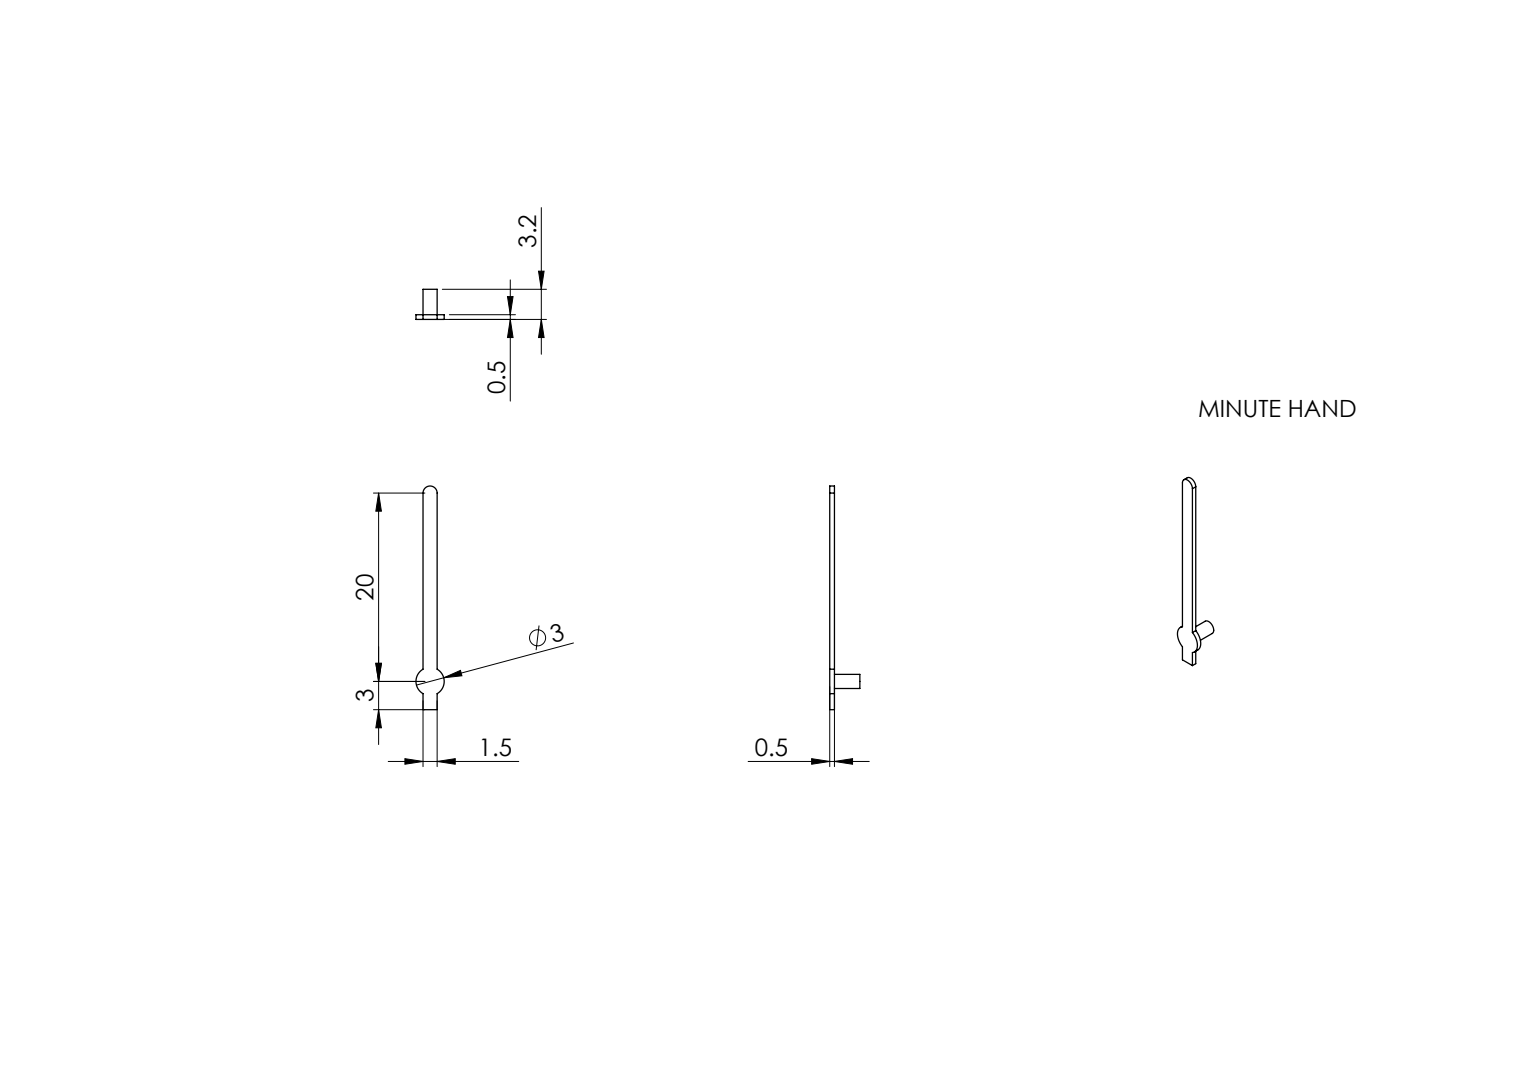
ISO-10303-21;
HEADER;
FILE_DESCRIPTION (('STEP AP214'),
    '1' );
FILE_NAME ('minute hand.step',
    '2026-10-26T11:20:31',
    ( '' ),
    ( '' ),
    'SwSTEP 2.0',
    'SolidWorks 2026',
    '' );
FILE_SCHEMA (( 'AUTOMOTIVE_DESIGN' ));
ENDSEC;

DATA;
#1=CARTESIAN_POINT ( 'NONE',  ( -0.7500000000000000000, 0.000000000000000000, 17.69999999999999929 ) ) ;
#7=ORIENTED_EDGE ( 'NONE', *, *, #1306, .T. ) ;
#18=DIRECTION ( 'NONE',  ( -0.000000000000000000, -0.000000000000000000, -1.000000000000000000 ) ) ;
#27=VERTEX_POINT ( 'NONE', #607 ) ;
#42=DIRECTION ( 'NONE',  ( 0.000000000000000000, 0.000000000000000000, 1.000000000000000000 ) ) ;
#70=ORIENTED_EDGE ( 'NONE', *, *, #687, .T. ) ;
#78=ORIENTED_EDGE ( 'NONE', *, *, #3001, .F. ) ;
#82=DIRECTION ( 'NONE',  ( 1.000000000000000000, 0.000000000000000000, 0.000000000000000000 ) ) ;
#87=LINE ( 'NONE', #2519, #444 ) ;
#97=CARTESIAN_POINT ( 'NONE',  ( 0.000000000000000000, 0.000000000000000000, 17.69999999999999929 ) ) ;
#113=ADVANCED_FACE ( 'NONE', ( #4266 ), #1343, .T. ) ;
#118=VECTOR ( 'NONE', #868, 1000.000000000000000 ) ;
#119=DIRECTION ( 'NONE',  ( 0.000000000000000000, 0.000000000000000000, 1.000000000000000000 ) ) ;
#140=DIRECTION ( 'NONE',  ( 0.000000000000000000, 0.000000000000000000, 1.000000000000000000 ) ) ;
#168=ORIENTED_EDGE ( 'NONE', *, *, #2422, .T. ) ;
#170=EDGE_LOOP ( 'NONE', ( #191, #1020, #400, #4142, #3752, #2488, #1167, #3281, #3139 ) ) ;
#183=DIRECTION ( 'NONE',  ( -1.000000000000000000, 0.000000000000000000, 0.000000000000000000 ) ) ;
#190=AXIS2_PLACEMENT_3D ( 'NONE', #1838, #4057, #3693 ) ;
#191=ORIENTED_EDGE ( 'NONE', *, *, #3421, .T. ) ;
#196=LINE ( 'NONE', #554, #4036 ) ;
#202=PLANE ( 'NONE',  #2959 ) ;
#256=FACE_OUTER_BOUND ( 'NONE', #2832, .T. ) ;
#258=ORIENTED_EDGE ( 'NONE', *, *, #4554, .T. ) ;
#260=AXIS2_PLACEMENT_3D ( 'NONE', #4512, #2060, #1677 ) ;
#292=CARTESIAN_POINT ( 'NONE',  ( -0.7500000000000001110, 20.00000000000000000, 18.19999999999999929 ) ) ;
#313=DIRECTION ( 'NONE',  ( 1.000000000000000000, 0.000000000000000000, 0.000000000000000000 ) ) ;
#316=DIRECTION ( 'NONE',  ( 0.000000000000000000, 0.000000000000000000, -1.000000000000000000 ) ) ;
#370=FACE_OUTER_BOUND ( 'NONE', #716, .T. ) ;
#386=ADVANCED_FACE ( 'NONE', ( #370 ), #2455, .F. ) ;
#396=DIRECTION ( 'NONE',  ( 1.000000000000000000, 0.000000000000000000, -0.000000000000000000 ) ) ;
#399=ORIENTED_EDGE ( 'NONE', *, *, #2054, .T. ) ;
#400=ORIENTED_EDGE ( 'NONE', *, *, #1846, .F. ) ;
#402=CARTESIAN_POINT ( 'NONE',  ( 0.7500000000000000000, -2.999999999999999556, 17.69999999999999929 ) ) ;
#416=FACE_OUTER_BOUND ( 'NONE', #1243, .T. ) ;
#419=CARTESIAN_POINT ( 'NONE',  ( 0.7500000000000001110, 1.299038105676658450, 17.69999999999999929 ) ) ;
#435=DIRECTION ( 'NONE',  ( -1.000000000000000000, 0.000000000000000000, -0.000000000000000000 ) ) ;
#443=ORIENTED_EDGE ( 'NONE', *, *, #2740, .F. ) ;
#444=VECTOR ( 'NONE', #4378, 1000.000000000000000 ) ;
#449=ORIENTED_EDGE ( 'NONE', *, *, #3217, .T. ) ;
#453=UNCERTAINTY_MEASURE_WITH_UNIT (LENGTH_MEASURE( 1.000000000000000082E-05 ), #1801, 'distance_accuracy_value', 'NONE');
#477=VERTEX_POINT ( 'NONE', #2505 ) ;
#478=ORIENTED_EDGE ( 'NONE', *, *, #3950, .F. ) ;
#482=LINE ( 'NONE', #3407, #3156 ) ;
#510=CARTESIAN_POINT ( 'NONE',  ( 0.7500000000000001110, 20.00000000000000000, 17.69999999999999929 ) ) ;
#511=LINE ( 'NONE', #1671, #1812 ) ;
#512=CARTESIAN_POINT ( 'NONE',  ( 0.000000000000000000, 20.00000000000000000, 17.69999999999999929 ) ) ;
#516=EDGE_CURVE ( 'NONE', #1550, #1737, #1460, .T. ) ;
#521=CARTESIAN_POINT ( 'NONE',  ( 0.7500000000000000000, -2.999999999999999556, 17.69999999999999929 ) ) ;
#524=ORIENTED_EDGE ( 'NONE', *, *, #4465, .F. ) ;
#541=CARTESIAN_POINT ( 'NONE',  ( 0.000000000000000000, 0.000000000000000000, 18.19999999999999929 ) ) ;
#544=DIRECTION ( 'NONE',  ( 0.000000000000000000, 0.000000000000000000, 1.000000000000000000 ) ) ;
#554=CARTESIAN_POINT ( 'NONE',  ( -0.7500000000000001110, 1.299038105676658450, 17.69999999999999929 ) ) ;
#556=ORIENTED_EDGE ( 'NONE', *, *, #1846, .T. ) ;
#562=ADVANCED_FACE ( 'NONE', ( #416 ), #2265, .T. ) ;
#566=AXIS2_PLACEMENT_3D ( 'NONE', #1204, #140, #4135 ) ;
#570=ORIENTED_EDGE ( 'NONE', *, *, #2926, .T. ) ;
#607=CARTESIAN_POINT ( 'NONE',  ( 0.7500000000000000000, -1.299038105676658450, 18.19999999999999929 ) ) ;
#635=CIRCLE ( 'NONE', #3283, 1.500000000000000222 ) ;
#658=VECTOR ( 'NONE', #781, 1000.000000000000000 ) ;
#677=CIRCLE ( 'NONE', #3941, 1.500000000000000222 ) ;
#678=DIRECTION ( 'NONE',  ( 0.000000000000000000, 0.000000000000000000, 1.000000000000000000 ) ) ;
#687=EDGE_CURVE ( 'NONE', #1161, #2307, #2576, .T. ) ;
#699=DIRECTION ( 'NONE',  ( 0.000000000000000000, 0.000000000000000000, 1.000000000000000000 ) ) ;
#714=DIRECTION ( 'NONE',  ( 0.000000000000000000, 0.000000000000000000, 1.000000000000000000 ) ) ;
#715=VERTEX_POINT ( 'NONE', #3488 ) ;
#716=EDGE_LOOP ( 'NONE', ( #908, #4000 ) ) ;
#720=ORIENTED_EDGE ( 'NONE', *, *, #4282, .F. ) ;
#723=DIRECTION ( 'NONE',  ( 0.000000000000000000, 0.000000000000000000, 1.000000000000000000 ) ) ;
#753=SHAPE_DEFINITION_REPRESENTATION ( #1564, #773 ) ;
#755=DIRECTION ( 'NONE',  ( -1.000000000000000000, 0.000000000000000000, 0.000000000000000000 ) ) ;
#756=CARTESIAN_POINT ( 'NONE',  ( 0.7500000000000001110, 9.184850993605150903E-17, 15.00000000000000178 ) ) ;
#765=VERTEX_POINT ( 'NONE', #1699 ) ;
#773=SHAPE_REPRESENTATION ( 'minute hand', ( #2928 ), #3769 ) ;
#774=FACE_OUTER_BOUND ( 'NONE', #4403, .T. ) ;
#781=DIRECTION ( 'NONE',  ( 0.000000000000000000, 0.000000000000000000, 1.000000000000000000 ) ) ;
#788=VERTEX_POINT ( 'NONE', #975 ) ;
#805=PLANE ( 'NONE',  #1597 ) ;
#809=CARTESIAN_POINT ( 'NONE',  ( -0.7500000000000001110, 20.00000000000000000, 17.69999999999999929 ) ) ;
#820=ADVANCED_FACE ( 'NONE', ( #2331 ), #3803, .T. ) ;
#837=UNCERTAINTY_MEASURE_WITH_UNIT (LENGTH_MEASURE( 1.000000000000000082E-05 ), #4288, 'distance_accuracy_value', 'NONE');
#848=AXIS2_PLACEMENT_3D ( 'NONE', #3084, #1630, #544 ) ;
#868=DIRECTION ( 'NONE',  ( -0.000000000000000000, -0.000000000000000000, -1.000000000000000000 ) ) ;
#908=ORIENTED_EDGE ( 'NONE', *, *, #3418, .F. ) ;
#911=DIRECTION ( 'NONE',  ( -0.000000000000000000, -0.000000000000000000, -1.000000000000000000 ) ) ;
#933=ORIENTED_EDGE ( 'NONE', *, *, #4502, .F. ) ;
#951=PLANE ( 'NONE',  #848 ) ;
#975=CARTESIAN_POINT ( 'NONE',  ( -0.7500000000000000000, -1.299038105676658450, 18.19999999999999929 ) ) ;
#990=DIRECTION ( 'NONE',  ( -0.000000000000000000, -1.000000000000000000, 0.000000000000000000 ) ) ;
#1000=ORIENTED_EDGE ( 'NONE', *, *, #3421, .F. ) ;
#1006=CIRCLE ( 'NONE', #3202, 1.500000000000000222 ) ;
#1018=LINE ( 'NONE', #3627, #2450 ) ;
#1020=ORIENTED_EDGE ( 'NONE', *, *, #3950, .T. ) ;
#1023=DIRECTION ( 'NONE',  ( -1.000000000000000000, 0.000000000000000000, 0.000000000000000000 ) ) ;
#1059=ADVANCED_FACE ( 'NONE', ( #2531 ), #3958, .T. ) ;
#1071=ORIENTED_EDGE ( 'NONE', *, *, #2422, .F. ) ;
#1096=CIRCLE ( 'NONE', #3147, 0.7500000000000001110 ) ;
#1126=CARTESIAN_POINT ( 'NONE',  ( 0.7500000000000001110, 1.299038105676658450, 17.69999999999999929 ) ) ;
#1161=VERTEX_POINT ( 'NONE', #809 ) ;
#1167=ORIENTED_EDGE ( 'NONE', *, *, #2110, .T. ) ;
#1203=ADVANCED_BREP_SHAPE_REPRESENTATION ( '', ( #1412, #2928 ), #3769 ) ;
#1204=CARTESIAN_POINT ( 'NONE',  ( 0.000000000000000000, 0.000000000000000000, 17.69999999999999929 ) ) ;
#1207=ORIENTED_EDGE ( 'NONE', *, *, #687, .F. ) ;
#1225=FACE_OUTER_BOUND ( 'NONE', #1963, .T. ) ;
#1226=CARTESIAN_POINT ( 'NONE',  ( 0.7500000000000001110, 9.184850993605150903E-17, 17.69999999999999929 ) ) ;
#1243=EDGE_LOOP ( 'NONE', ( #4067, #570, #933, #1367 ) ) ;
#1261=AXIS2_PLACEMENT_3D ( 'NONE', #2615, #3685, #2908 ) ;
#1270=VERTEX_POINT ( 'NONE', #4177 ) ;
#1273=VECTOR ( 'NONE', #3225, 1000.000000000000000 ) ;
#1278=DIRECTION ( 'NONE',  ( -0.000000000000000000, -1.000000000000000000, -0.000000000000000000 ) ) ;
#1295=LINE ( 'NONE', #3165, #2483 ) ;
#1299=EDGE_LOOP ( 'NONE', ( #1806, #4350, #399, #3813 ) ) ;
#1306=EDGE_CURVE ( 'NONE', #715, #1870, #196, .T. ) ;
#1320=SURFACE_STYLE_USAGE ( .BOTH. , #3761 ) ;
#1323=DIRECTION ( 'NONE',  ( 0.000000000000000000, 0.000000000000000000, 1.000000000000000000 ) ) ;
#1326=LINE ( 'NONE', #2372, #1627 ) ;
#1342=VECTOR ( 'NONE', #3381, 1000.000000000000000 ) ;
#1343=PLANE ( 'NONE',  #4188 ) ;
#1358=ORIENTED_EDGE ( 'NONE', *, *, #4137, .F. ) ;
#1367=ORIENTED_EDGE ( 'NONE', *, *, #4282, .T. ) ;
#1369=DIRECTION ( 'NONE',  ( -0.000000000000000000, -1.000000000000000000, 0.000000000000000000 ) ) ;
#1372=LINE ( 'NONE', #3247, #2978 ) ;
#1412=MANIFOLD_SOLID_BREP ( 'Extrude-Thin1', #2143 ) ;
#1445=( NAMED_UNIT ( * ) PLANE_ANGLE_UNIT ( ) SI_UNIT ( $, .RADIAN. ) );
#1460=LINE ( 'NONE', #1, #1273 ) ;
#1508=ORIENTED_EDGE ( 'NONE', *, *, #3086, .T. ) ;
#1526=ADVANCED_FACE ( 'NONE', ( #4069, #1823 ), #805, .F. ) ;
#1541=EDGE_LOOP ( 'NONE', ( #3473, #2533, #2637, #3666 ) ) ;
#1544=ORIENTED_EDGE ( 'NONE', *, *, #2306, .T. ) ;
#1550=VERTEX_POINT ( 'NONE', #1847 ) ;
#1560=VERTEX_POINT ( 'NONE', #419 ) ;
#1564=PRODUCT_DEFINITION_SHAPE ( 'NONE', 'NONE',  #3507 ) ;
#1570=ORIENTED_EDGE ( 'NONE', *, *, #516, .T. ) ;
#1590=ORIENTED_EDGE ( 'NONE', *, *, #2926, .F. ) ;
#1597=AXIS2_PLACEMENT_3D ( 'NONE', #97, #119, #396 ) ;
#1606=VECTOR ( 'NONE', #2974, 1000.000000000000000 ) ;
#1627=VECTOR ( 'NONE', #1278, 1000.000000000000000 ) ;
#1630=DIRECTION ( 'NONE',  ( 0.000000000000000000, 1.000000000000000000, -0.000000000000000000 ) ) ;
#1631=DIRECTION ( 'NONE',  ( 0.000000000000000000, 0.000000000000000000, 1.000000000000000000 ) ) ;
#1638=CARTESIAN_POINT ( 'NONE',  ( -0.7500000000000001110, 0.000000000000000000, 18.19999999999999929 ) ) ;
#1648=DIRECTION ( 'NONE',  ( 0.000000000000000000, 0.000000000000000000, 1.000000000000000000 ) ) ;
#1665=LINE ( 'NONE', #2004, #1342 ) ;
#1669=CARTESIAN_POINT ( 'NONE',  ( 0.000000000000000000, 0.000000000000000000, 17.69999999999999929 ) ) ;
#1670=ADVANCED_FACE ( 'NONE', ( #4567 ), #951, .F. ) ;
#1671=CARTESIAN_POINT ( 'NONE',  ( -0.7500000000000000000, -2.999999999999999556, 17.69999999999999929 ) ) ;
#1677=DIRECTION ( 'NONE',  ( -0.000000000000000000, 0.000000000000000000, 1.000000000000000000 ) ) ;
#1680=CYLINDRICAL_SURFACE ( 'NONE', #3112, 1.500000000000000222 ) ;
#1697=CARTESIAN_POINT ( 'NONE',  ( 0.7500000000000001110, 0.000000000000000000, 17.69999999999999929 ) ) ;
#1699=CARTESIAN_POINT ( 'NONE',  ( 0.7500000000000001110, 1.299038105676658450, 18.19999999999999929 ) ) ;
#1705=DIRECTION ( 'NONE',  ( 0.000000000000000000, 0.000000000000000000, 1.000000000000000000 ) ) ;
#1712=DIRECTION ( 'NONE',  ( 0.000000000000000000, 0.000000000000000000, 1.000000000000000000 ) ) ;
#1737=VERTEX_POINT ( 'NONE', #3177 ) ;
#1738=DIRECTION ( 'NONE',  ( 1.000000000000000000, 0.000000000000000000, -0.000000000000000000 ) ) ;
#1739=CARTESIAN_POINT ( 'NONE',  ( 0.000000000000000000, 0.000000000000000000, 17.69999999999999929 ) ) ;
#1753=DIRECTION ( 'NONE',  ( 1.000000000000000000, 0.000000000000000000, -0.000000000000000000 ) ) ;
#1767=CIRCLE ( 'NONE', #3822, 0.7500000000000001110 ) ;
#1768=EDGE_CURVE ( 'NONE', #4595, #1560, #1006, .T. ) ;
#1780=CARTESIAN_POINT ( 'NONE',  ( 0.000000000000000000, 0.000000000000000000, 0.000000000000000000 ) ) ;
#1786=CARTESIAN_POINT ( 'NONE',  ( 0.7500000000000000000, 0.000000000000000000, 18.19999999999999929 ) ) ;
#1801=( LENGTH_UNIT ( ) NAMED_UNIT ( * ) SI_UNIT ( .MILLI., .METRE. ) );
#1806=ORIENTED_EDGE ( 'NONE', *, *, #1935, .F. ) ;
#1812=VECTOR ( 'NONE', #2741, 1000.000000000000000 ) ;
#1820=EDGE_LOOP ( 'NONE', ( #556, #2302, #1358, #168 ) ) ;
#1822=ORIENTED_EDGE ( 'NONE', *, *, #4059, .F. ) ;
#1823=FACE_BOUND ( 'NONE', #4209, .T. ) ;
#1838=CARTESIAN_POINT ( 'NONE',  ( 0.000000000000000000, 0.000000000000000000, 18.19999999999999929 ) ) ;
#1846=EDGE_CURVE ( 'NONE', #3324, #477, #1372, .T. ) ;
#1847=CARTESIAN_POINT ( 'NONE',  ( -0.7500000000000000000, -1.299038105676658450, 17.69999999999999929 ) ) ;
#1870=VERTEX_POINT ( 'NONE', #4038 ) ;
#1886=DIRECTION ( 'NONE',  ( -0.000000000000000000, 0.000000000000000000, 1.000000000000000000 ) ) ;
#1918=VECTOR ( 'NONE', #3458, 1000.000000000000000 ) ;
#1934=ORIENTED_EDGE ( 'NONE', *, *, #2690, .F. ) ;
#1935=EDGE_CURVE ( 'NONE', #1560, #765, #2953, .T. ) ;
#1962=DIRECTION ( 'NONE',  ( -0.000000000000000000, -0.000000000000000000, -1.000000000000000000 ) ) ;
#1963=EDGE_LOOP ( 'NONE', ( #3306, #1934, #1207, #4237 ) ) ;
#1984=LINE ( 'NONE', #2006, #1918 ) ;
#1990=DIRECTION ( 'NONE',  ( -0.000000000000000000, -0.000000000000000000, -1.000000000000000000 ) ) ;
#2001=CARTESIAN_POINT ( 'NONE',  ( 0.000000000000000000, 0.000000000000000000, 18.19999999999999929 ) ) ;
#2004=CARTESIAN_POINT ( 'NONE',  ( 0.7500000000000001110, 0.000000000000000000, 17.69999999999999929 ) ) ;
#2006=CARTESIAN_POINT ( 'NONE',  ( 0.7500000000000001110, 0.000000000000000000, 18.19999999999999929 ) ) ;
#2008=CARTESIAN_POINT ( 'NONE',  ( -0.7500000000000001110, 0.000000000000000000, 15.00000000000000178 ) ) ;
#2033=PRODUCT_DEFINITION_FORMATION_WITH_SPECIFIED_SOURCE ( 'ANY', '', #2787, .NOT_KNOWN. ) ;
#2048=DIRECTION ( 'NONE',  ( -0.000000000000000000, -0.000000000000000000, -1.000000000000000000 ) ) ;
#2054=EDGE_CURVE ( 'NONE', #2878, #1270, #2643, .T. ) ;
#2060=DIRECTION ( 'NONE',  ( -1.000000000000000000, 0.000000000000000000, -0.000000000000000000 ) ) ;
#2069=CYLINDRICAL_SURFACE ( 'NONE', #4016, 0.7500000000000001110 ) ;
#2071=( NAMED_UNIT ( * ) PLANE_ANGLE_UNIT ( ) SI_UNIT ( $, .RADIAN. ) );
#2079=LINE ( 'NONE', #2401, #3946 ) ;
#2080=CARTESIAN_POINT ( 'NONE',  ( -0.7500000000000000000, 0.000000000000000000, 18.19999999999999929 ) ) ;
#2110=EDGE_CURVE ( 'NONE', #765, #1270, #1984, .T. ) ;
#2123=CIRCLE ( 'NONE', #4319, 0.7500000000000001110 ) ;
#2138=DIRECTION ( 'NONE',  ( 1.000000000000000000, 0.000000000000000000, 0.000000000000000000 ) ) ;
#2143=CLOSED_SHELL ( 'NONE', ( #820, #562, #3805, #2749, #113, #386, #1526, #3104, #1059, #2895, #3414, #2984, #3887, #1670 ) ) ;
#2145=LINE ( 'NONE', #402, #3166 ) ;
#2153=CARTESIAN_POINT ( 'NONE',  ( 0.000000000000000000, 20.00000000000000000, 18.19999999999999929 ) ) ;
#2214=EDGE_CURVE ( 'NONE', #4100, #4120, #1767, .T. ) ;
#2231=CARTESIAN_POINT ( 'NONE',  ( 0.000000000000000000, 0.000000000000000000, 18.19999999999999929 ) ) ;
#2234=CIRCLE ( 'NONE', #2848, 1.500000000000000222 ) ;
#2253=ORIENTED_EDGE ( 'NONE', *, *, #2054, .F. ) ;
#2261=CARTESIAN_POINT ( 'NONE',  ( 0.7500000000000000000, -2.999999999999999556, 17.69999999999999929 ) ) ;
#2262=AXIS2_PLACEMENT_3D ( 'NONE', #1697, #3573, #316 ) ;
#2265=CYLINDRICAL_SURFACE ( 'NONE', #2857, 1.500000000000000222 ) ;
#2302=ORIENTED_EDGE ( 'NONE', *, *, #3086, .F. ) ;
#2306=EDGE_CURVE ( 'NONE', #1870, #1550, #2981, .T. ) ;
#2307=VERTEX_POINT ( 'NONE', #292 ) ;
#2316=EDGE_LOOP ( 'NONE', ( #2732, #3638, #3020, #4066, #3679, #2871, #3812, #3526, #2804 ) ) ;
#2323=DIRECTION ( 'NONE',  ( 0.000000000000000000, 0.000000000000000000, 1.000000000000000000 ) ) ;
#2327=AXIS2_PLACEMENT_3D ( 'NONE', #3982, #723, #4124 ) ;
#2331=FACE_OUTER_BOUND ( 'NONE', #1541, .T. ) ;
#2349=ORIENTED_EDGE ( 'NONE', *, *, #2214, .T. ) ;
#2352=EDGE_CURVE ( 'NONE', #4496, #4595, #635, .T. ) ;
#2358=CARTESIAN_POINT ( 'NONE',  ( 0.000000000000000000, 0.000000000000000000, 18.19999999999999929 ) ) ;
#2364=ORIENTED_EDGE ( 'NONE', *, *, #3418, .T. ) ;
#2372=CARTESIAN_POINT ( 'NONE',  ( -0.7500000000000001110, 0.000000000000000000, 17.69999999999999929 ) ) ;
#2401=CARTESIAN_POINT ( 'NONE',  ( 1.500000000000000222, 0.000000000000000000, 17.69999999999999929 ) ) ;
#2422=EDGE_CURVE ( 'NONE', #3310, #3324, #2145, .T. ) ;
#2440=DIRECTION ( 'NONE',  ( 0.000000000000000000, 0.000000000000000000, 1.000000000000000000 ) ) ;
#2446=APPLICATION_CONTEXT ( 'automotive_design' ) ;
#2450=VECTOR ( 'NONE', #18, 1000.000000000000000 ) ;
#2455=PLANE ( 'NONE',  #3311 ) ;
#2459=DIRECTION ( 'NONE',  ( -0.000000000000000000, -1.000000000000000000, -0.000000000000000000 ) ) ;
#2464=CARTESIAN_POINT ( 'NONE',  ( 0.000000000000000000, 0.000000000000000000, 18.19999999999999929 ) ) ;
#2472=LINE ( 'NONE', #2080, #3905 ) ;
#2483=VECTOR ( 'NONE', #2048, 1000.000000000000000 ) ;
#2488=ORIENTED_EDGE ( 'NONE', *, *, #4059, .T. ) ;
#2505=CARTESIAN_POINT ( 'NONE',  ( -0.7500000000000000000, -2.999999999999999556, 18.19999999999999929 ) ) ;
#2509=STYLED_ITEM('',(#4736),#1412);
#2515=APPLICATION_CONTEXT ( 'automotive_design' ) ;
#2519=CARTESIAN_POINT ( 'NONE',  ( 0.7500000000000000000, 0.000000000000000000, 17.69999999999999929 ) ) ;
#2531=FACE_OUTER_BOUND ( 'NONE', #3786, .T. ) ;
#2533=ORIENTED_EDGE ( 'NONE', *, *, #2740, .T. ) ;
#2537=EDGE_CURVE ( 'NONE', #3687, #4371, #3944, .T. ) ;
#2576=LINE ( 'NONE', #4040, #658 ) ;
#2602=CARTESIAN_POINT ( 'NONE',  ( 0.000000000000000000, 0.000000000000000000, 17.69999999999999929 ) ) ;
#2603=ORIENTED_EDGE ( 'NONE', *, *, #1768, .T. ) ;
#2615=CARTESIAN_POINT ( 'NONE',  ( 0.000000000000000000, 0.000000000000000000, 17.69999999999999929 ) ) ;
#2624=FACE_OUTER_BOUND ( 'NONE', #4675, .T. ) ;
#2637=ORIENTED_EDGE ( 'NONE', *, *, #2537, .T. ) ;
#2643=LINE ( 'NONE', #510, #2825 ) ;
#2683=FILL_AREA_STYLE ('',( #3985 ) ) ;
#2690=EDGE_CURVE ( 'NONE', #2307, #715, #3814, .T. ) ;
#2692=CARTESIAN_POINT ( 'NONE',  ( 0.7500000000000000000, -1.299038105676658450, 17.69999999999999929 ) ) ;
#2712=( NAMED_UNIT ( * ) PLANE_ANGLE_UNIT ( ) SI_UNIT ( $, .RADIAN. ) );
#2718=VECTOR ( 'NONE', #990, 1000.000000000000000 ) ;
#2732=ORIENTED_EDGE ( 'NONE', *, *, #2352, .F. ) ;
#2735=DIRECTION ( 'NONE',  ( -0.000000000000000000, -0.000000000000000000, -1.000000000000000000 ) ) ;
#2740=EDGE_CURVE ( 'NONE', #4100, #3687, #1295, .T. ) ;
#2741=DIRECTION ( 'NONE',  ( 0.000000000000000000, 0.000000000000000000, 1.000000000000000000 ) ) ;
#2749=ADVANCED_FACE ( 'NONE', ( #3496 ), #2069, .T. ) ;
#2764=CARTESIAN_POINT ( 'NONE',  ( -0.7500000000000001110, 0.000000000000000000, 17.69999999999999929 ) ) ;
#2775=DIRECTION ( 'NONE',  ( 1.000000000000000000, 0.000000000000000000, 0.000000000000000000 ) ) ;
#2787=PRODUCT ( 'minute hand', 'minute hand', '', ( #4688 ) ) ;
#2804=ORIENTED_EDGE ( 'NONE', *, *, #1768, .F. ) ;
#2825=VECTOR ( 'NONE', #2323, 1000.000000000000000 ) ;
#2832=EDGE_LOOP ( 'NONE', ( #4409, #1000, #7, #1544 ) ) ;
#2835=LINE ( 'NONE', #1786, #2718 ) ;
#2848=AXIS2_PLACEMENT_3D ( 'NONE', #2231, #4458, #82 ) ;
#2849=VERTEX_POINT ( 'NONE', #4574 ) ;
#2856=MECHANICAL_DESIGN_GEOMETRIC_PRESENTATION_REPRESENTATION('',(#3921),#3688);
#2857=AXIS2_PLACEMENT_3D ( 'NONE', #2602, #42, #3317 ) ;
#2863=CARTESIAN_POINT ( 'NONE',  ( 0.7500000000000001110, 20.00000000000000000, 17.69999999999999929 ) ) ;
#2868=DIRECTION ( 'NONE',  ( 1.000000000000000000, 0.000000000000000000, 0.000000000000000000 ) ) ;
#2871=ORIENTED_EDGE ( 'NONE', *, *, #4271, .F. ) ;
#2878=VERTEX_POINT ( 'NONE', #2863 ) ;
#2895=ADVANCED_FACE ( 'NONE', ( #3940 ), #3889, .T. ) ;
#2908=DIRECTION ( 'NONE',  ( 1.000000000000000000, 0.000000000000000000, 0.000000000000000000 ) ) ;
#2926=EDGE_CURVE ( 'NONE', #4595, #2849, #2079, .T. ) ;
#2928=AXIS2_PLACEMENT_3D ( 'NONE', #1780, #1712, #3957 ) ;
#2953=LINE ( 'NONE', #1126, #1606 ) ;
#2959=AXIS2_PLACEMENT_3D ( 'NONE', #2764, #3818, #1648 ) ;
#2974=DIRECTION ( 'NONE',  ( 0.000000000000000000, 0.000000000000000000, 1.000000000000000000 ) ) ;
#2978=VECTOR ( 'NONE', #755, 1000.000000000000000 ) ;
#2981=CIRCLE ( 'NONE', #4210, 1.500000000000000222 ) ;
#2982=LINE ( 'NONE', #2261, #3000 ) ;
#2984=ADVANCED_FACE ( 'NONE', ( #774 ), #3690, .T. ) ;
#3000=VECTOR ( 'NONE', #3363, 1000.000000000000000 ) ;
#3001=EDGE_CURVE ( 'NONE', #4496, #3310, #87, .T. ) ;
#3007=COLOUR_RGB ( '',0.8941176470588234615, 0.8941176470588234615, 0.8941176470588234615 ) ;
#3020=ORIENTED_EDGE ( 'NONE', *, *, #4137, .T. ) ;
#3037=CARTESIAN_POINT ( 'NONE',  ( 0.7500000000000000000, -2.999999999999999556, 18.19999999999999929 ) ) ;
#3058=FACE_OUTER_BOUND ( 'NONE', #4632, .T. ) ;
#3084=CARTESIAN_POINT ( 'NONE',  ( 0.7500000000000000000, -2.999999999999999556, 17.69999999999999929 ) ) ;
#3086=EDGE_CURVE ( 'NONE', #1737, #477, #511, .T. ) ;
#3089=AXIS2_PLACEMENT_3D ( 'NONE', #541, #1990, #183 ) ;
#3091=ORIENTED_EDGE ( 'NONE', *, *, #1935, .T. ) ;
#3104=ADVANCED_FACE ( 'NONE', ( #1225 ), #202, .T. ) ;
#3112=AXIS2_PLACEMENT_3D ( 'NONE', #3158, #4215, #2775 ) ;
#3125=LINE ( 'NONE', #2692, #118 ) ;
#3139=ORIENTED_EDGE ( 'NONE', *, *, #2690, .T. ) ;
#3147=AXIS2_PLACEMENT_3D ( 'NONE', #2153, #4015, #2868 ) ;
#3153=CIRCLE ( 'NONE', #190, 1.500000000000000222 ) ;
#3156=VECTOR ( 'NONE', #1962, 1000.000000000000000 ) ;
#3157=CARTESIAN_POINT ( 'NONE',  ( 0.000000000000000000, 0.000000000000000000, 17.69999999999999929 ) ) ;
#3158=CARTESIAN_POINT ( 'NONE',  ( 0.000000000000000000, 0.000000000000000000, 17.69999999999999929 ) ) ;
#3165=CARTESIAN_POINT ( 'NONE',  ( 0.7500000000000001110, 9.184850993605150903E-17, 18.19999999999999929 ) ) ;
#3166=VECTOR ( 'NONE', #4677, 1000.000000000000000 ) ;
#3177=CARTESIAN_POINT ( 'NONE',  ( -0.7500000000000000000, -2.999999999999999556, 17.69999999999999929 ) ) ;
#3202=AXIS2_PLACEMENT_3D ( 'NONE', #3157, #4255, #3223 ) ;
#3217=EDGE_CURVE ( 'NONE', #27, #3324, #2835, .T. ) ;
#3223=DIRECTION ( 'NONE',  ( 1.000000000000000000, 0.000000000000000000, 0.000000000000000000 ) ) ;
#3225=DIRECTION ( 'NONE',  ( -0.000000000000000000, -1.000000000000000000, 0.000000000000000000 ) ) ;
#3247=CARTESIAN_POINT ( 'NONE',  ( 0.7500000000000000000, -2.999999999999999556, 18.19999999999999929 ) ) ;
#3268=( GEOMETRIC_REPRESENTATION_CONTEXT ( 3 ) GLOBAL_UNCERTAINTY_ASSIGNED_CONTEXT ( ( #837 ) ) GLOBAL_UNIT_ASSIGNED_CONTEXT ( ( #4288, #2071, #3953 ) ) REPRESENTATION_CONTEXT ( 'NONE', 'WORKASPACE' ) );
#3280=EDGE_LOOP ( 'NONE', ( #443, #524, #4080, #2364 ) ) ;
#3281=ORIENTED_EDGE ( 'NONE', *, *, #3595, .T. ) ;
#3283=AXIS2_PLACEMENT_3D ( 'NONE', #1669, #1323, #3904 ) ;
#3295=ORIENTED_EDGE ( 'NONE', *, *, #3595, .F. ) ;
#3306=ORIENTED_EDGE ( 'NONE', *, *, #1306, .F. ) ;
#3310=VERTEX_POINT ( 'NONE', #521 ) ;
#3311=AXIS2_PLACEMENT_3D ( 'NONE', #4306, #714, #1753 ) ;
#3317=DIRECTION ( 'NONE',  ( 1.000000000000000000, 0.000000000000000000, 0.000000000000000000 ) ) ;
#3324=VERTEX_POINT ( 'NONE', #3037 ) ;
#3363=DIRECTION ( 'NONE',  ( -1.000000000000000000, 0.000000000000000000, 0.000000000000000000 ) ) ;
#3376=ORIENTED_EDGE ( 'NONE', *, *, #4465, .T. ) ;
#3381=DIRECTION ( 'NONE',  ( 0.000000000000000000, 1.000000000000000000, 0.000000000000000000 ) ) ;
#3394=CYLINDRICAL_SURFACE ( 'NONE', #566, 1.500000000000000222 ) ;
#3407=CARTESIAN_POINT ( 'NONE',  ( -0.7500000000000000000, -1.299038105676658450, 17.69999999999999929 ) ) ;
#3412=DIRECTION ( 'NONE',  ( 0.000000000000000000, 0.000000000000000000, 1.000000000000000000 ) ) ;
#3414=ADVANCED_FACE ( 'NONE', ( #256 ), #1680, .T. ) ;
#3418=EDGE_CURVE ( 'NONE', #4371, #3687, #2123, .T. ) ;
#3421=EDGE_CURVE ( 'NONE', #715, #788, #677, .T. ) ;
#3458=DIRECTION ( 'NONE',  ( 0.000000000000000000, 1.000000000000000000, 0.000000000000000000 ) ) ;
#3473=ORIENTED_EDGE ( 'NONE', *, *, #2214, .F. ) ;
#3481=DIRECTION ( 'NONE',  ( 1.000000000000000000, 0.000000000000000000, 0.000000000000000000 ) ) ;
#3488=CARTESIAN_POINT ( 'NONE',  ( -0.7500000000000001110, 1.299038105676658450, 18.19999999999999929 ) ) ;
#3490=CARTESIAN_POINT ( 'NONE',  ( 0.000000000000000000, 0.000000000000000000, 15.00000000000000178 ) ) ;
#3496=FACE_OUTER_BOUND ( 'NONE', #3280, .T. ) ;
#3500=CARTESIAN_POINT ( 'NONE',  ( 0.000000000000000000, 0.000000000000000000, 17.69999999999999929 ) ) ;
#3507=PRODUCT_DEFINITION ( 'UNKNOWN', '', #2033, #4626 ) ;
#3526=ORIENTED_EDGE ( 'NONE', *, *, #4622, .F. ) ;
#3573=DIRECTION ( 'NONE',  ( 1.000000000000000000, 0.000000000000000000, 0.000000000000000000 ) ) ;
#3595=EDGE_CURVE ( 'NONE', #1270, #2307, #1096, .T. ) ;
#3622=EDGE_CURVE ( 'NONE', #4120, #4371, #1018, .T. ) ;
#3627=CARTESIAN_POINT ( 'NONE',  ( -0.7500000000000001110, 0.000000000000000000, 18.19999999999999929 ) ) ;
#3638=ORIENTED_EDGE ( 'NONE', *, *, #3001, .T. ) ;
#3644=CARTESIAN_POINT ( 'NONE',  ( -0.7500000000000000000, 0.000000000000000000, 17.69999999999999929 ) ) ;
#3647=MECHANICAL_DESIGN_GEOMETRIC_PRESENTATION_REPRESENTATION('',(#2509),#3268);
#3666=ORIENTED_EDGE ( 'NONE', *, *, #3622, .F. ) ;
#3677=CIRCLE ( 'NONE', #1261, 0.7500000000000001110 ) ;
#3679=ORIENTED_EDGE ( 'NONE', *, *, #2306, .F. ) ;
#3685=DIRECTION ( 'NONE',  ( 0.000000000000000000, 0.000000000000000000, 1.000000000000000000 ) ) ;
#3687=VERTEX_POINT ( 'NONE', #756 ) ;
#3688=( GEOMETRIC_REPRESENTATION_CONTEXT ( 3 ) GLOBAL_UNCERTAINTY_ASSIGNED_CONTEXT ( ( #3732 ) ) GLOBAL_UNIT_ASSIGNED_CONTEXT ( ( #4126, #2712, #4179 ) ) REPRESENTATION_CONTEXT ( 'NONE', 'WORKASPACE' ) );
#3690=PLANE ( 'NONE',  #4555 ) ;
#3693=DIRECTION ( 'NONE',  ( 1.000000000000000000, 0.000000000000000000, 0.000000000000000000 ) ) ;
#3732=UNCERTAINTY_MEASURE_WITH_UNIT (LENGTH_MEASURE( 1.000000000000000082E-05 ), #4126, 'distance_accuracy_value', 'NONE');
#3752=ORIENTED_EDGE ( 'NONE', *, *, #4502, .T. ) ;
#3761=SURFACE_SIDE_STYLE ('',( #4598 ) ) ;
#3769=( GEOMETRIC_REPRESENTATION_CONTEXT ( 3 ) GLOBAL_UNCERTAINTY_ASSIGNED_CONTEXT ( ( #453 ) ) GLOBAL_UNIT_ASSIGNED_CONTEXT ( ( #1801, #1445, #4353 ) ) REPRESENTATION_CONTEXT ( 'NONE', 'WORKASPACE' ) );
#3786=EDGE_LOOP ( 'NONE', ( #3295, #2253, #4454, #70 ) ) ;
#3802=PLANE ( 'NONE',  #260 ) ;
#3803=CYLINDRICAL_SURFACE ( 'NONE', #3089, 0.7500000000000001110 ) ;
#3805=ADVANCED_FACE ( 'NONE', ( #2624 ), #3394, .T. ) ;
#3812=ORIENTED_EDGE ( 'NONE', *, *, #4301, .F. ) ;
#3813=ORIENTED_EDGE ( 'NONE', *, *, #2110, .F. ) ;
#3814=LINE ( 'NONE', #1638, #4630 ) ;
#3818=DIRECTION ( 'NONE',  ( -1.000000000000000000, 0.000000000000000000, 0.000000000000000000 ) ) ;
#3822=AXIS2_PLACEMENT_3D ( 'NONE', #3500, #2440, #4603 ) ;
#3887=ADVANCED_FACE ( 'NONE', ( #3058 ), #3802, .F. ) ;
#3889=PLANE ( 'NONE',  #2262 ) ;
#3904=DIRECTION ( 'NONE',  ( 1.000000000000000000, 0.000000000000000000, 0.000000000000000000 ) ) ;
#3905=VECTOR ( 'NONE', #1369, 1000.000000000000000 ) ;
#3921=STYLED_ITEM ( 'NONE', ( #4504 ), #1203 ) ;
#3940=FACE_OUTER_BOUND ( 'NONE', #1299, .T. ) ;
#3941=AXIS2_PLACEMENT_3D ( 'NONE', #2358, #1705, #4616 ) ;
#3944=CIRCLE ( 'NONE', #2327, 0.7500000000000001110 ) ;
#3946=VECTOR ( 'NONE', #4608, 1000.000000000000000 ) ;
#3950=EDGE_CURVE ( 'NONE', #788, #477, #2472, .T. ) ;
#3953=( NAMED_UNIT ( * ) SI_UNIT ( $, .STERADIAN. ) SOLID_ANGLE_UNIT ( ) );
#3957=DIRECTION ( 'NONE',  ( 1.000000000000000000, 0.000000000000000000, 0.000000000000000000 ) ) ;
#3958=CYLINDRICAL_SURFACE ( 'NONE', #3961, 0.7500000000000001110 ) ;
#3961=AXIS2_PLACEMENT_3D ( 'NONE', #3999, #699, #2138 ) ;
#3982=CARTESIAN_POINT ( 'NONE',  ( 0.000000000000000000, 0.000000000000000000, 15.00000000000000178 ) ) ;
#3985=FILL_AREA_STYLE_COLOUR ( '', #3007 ) ;
#3999=CARTESIAN_POINT ( 'NONE',  ( 0.000000000000000000, 20.00000000000000000, 17.69999999999999929 ) ) ;
#4000=ORIENTED_EDGE ( 'NONE', *, *, #2537, .F. ) ;
#4015=DIRECTION ( 'NONE',  ( 0.000000000000000000, 0.000000000000000000, 1.000000000000000000 ) ) ;
#4016=AXIS2_PLACEMENT_3D ( 'NONE', #2001, #2735, #1023 ) ;
#4036=VECTOR ( 'NONE', #911, 1000.000000000000000 ) ;
#4038=CARTESIAN_POINT ( 'NONE',  ( -0.7500000000000001110, 1.299038105676658450, 17.69999999999999929 ) ) ;
#4040=CARTESIAN_POINT ( 'NONE',  ( -0.7500000000000001110, 20.00000000000000000, 17.69999999999999929 ) ) ;
#4057=DIRECTION ( 'NONE',  ( 0.000000000000000000, 0.000000000000000000, 1.000000000000000000 ) ) ;
#4059=EDGE_CURVE ( 'NONE', #2849, #765, #3153, .T. ) ;
#4066=ORIENTED_EDGE ( 'NONE', *, *, #516, .F. ) ;
#4067=ORIENTED_EDGE ( 'NONE', *, *, #2352, .T. ) ;
#4069=FACE_OUTER_BOUND ( 'NONE', #2316, .T. ) ;
#4080=ORIENTED_EDGE ( 'NONE', *, *, #3622, .T. ) ;
#4085=CARTESIAN_POINT ( 'NONE',  ( -0.7500000000000001110, 0.000000000000000000, 17.69999999999999929 ) ) ;
#4100=VERTEX_POINT ( 'NONE', #1226 ) ;
#4120=VERTEX_POINT ( 'NONE', #4085 ) ;
#4124=DIRECTION ( 'NONE',  ( 1.000000000000000000, 0.000000000000000000, 0.000000000000000000 ) ) ;
#4126=( LENGTH_UNIT ( ) NAMED_UNIT ( * ) SI_UNIT ( .MILLI., .METRE. ) );
#4135=DIRECTION ( 'NONE',  ( 1.000000000000000000, 0.000000000000000000, 0.000000000000000000 ) ) ;
#4137=EDGE_CURVE ( 'NONE', #3310, #1737, #2982, .T. ) ;
#4142=ORIENTED_EDGE ( 'NONE', *, *, #3217, .F. ) ;
#4151=SHAPE_REPRESENTATION_RELATIONSHIP ( 'NONE' , 'NONE' ,  #773, #1203 ) ;
#4177=CARTESIAN_POINT ( 'NONE',  ( 0.7500000000000001110, 20.00000000000000000, 18.19999999999999929 ) ) ;
#4179=( NAMED_UNIT ( * ) SI_UNIT ( $, .STERADIAN. ) SOLID_ANGLE_UNIT ( ) );
#4180=CARTESIAN_POINT ( 'NONE',  ( 1.500000000000000222, 0.000000000000000000, 17.69999999999999929 ) ) ;
#4188=AXIS2_PLACEMENT_3D ( 'NONE', #2464, #4627, #1738 ) ;
#4209=EDGE_LOOP ( 'NONE', ( #3376, #2349 ) ) ;
#4210=AXIS2_PLACEMENT_3D ( 'NONE', #1739, #678, #313 ) ;
#4215=DIRECTION ( 'NONE',  ( 0.000000000000000000, 0.000000000000000000, 1.000000000000000000 ) ) ;
#4237=ORIENTED_EDGE ( 'NONE', *, *, #4271, .T. ) ;
#4255=DIRECTION ( 'NONE',  ( 0.000000000000000000, 0.000000000000000000, 1.000000000000000000 ) ) ;
#4266=FACE_OUTER_BOUND ( 'NONE', #170, .T. ) ;
#4271=EDGE_CURVE ( 'NONE', #1161, #1870, #1326, .T. ) ;
#4282=EDGE_CURVE ( 'NONE', #27, #4496, #3125, .T. ) ;
#4288=( LENGTH_UNIT ( ) NAMED_UNIT ( * ) SI_UNIT ( .MILLI., .METRE. ) );
#4297=CIRCLE ( 'NONE', #4682, 0.7500000000000001110 ) ;
#4301=EDGE_CURVE ( 'NONE', #2878, #1161, #4297, .T. ) ;
#4306=CARTESIAN_POINT ( 'NONE',  ( 0.000000000000000000, 0.000000000000000000, 15.00000000000000178 ) ) ;
#4319=AXIS2_PLACEMENT_3D ( 'NONE', #3490, #1631, #4591 ) ;
#4350=ORIENTED_EDGE ( 'NONE', *, *, #4622, .T. ) ;
#4353=( NAMED_UNIT ( * ) SI_UNIT ( $, .STERADIAN. ) SOLID_ANGLE_UNIT ( ) );
#4371=VERTEX_POINT ( 'NONE', #2008 ) ;
#4378=DIRECTION ( 'NONE',  ( -0.000000000000000000, -1.000000000000000000, 0.000000000000000000 ) ) ;
#4403=EDGE_LOOP ( 'NONE', ( #478, #258, #1570, #1508 ) ) ;
#4407=CARTESIAN_POINT ( 'NONE',  ( 0.7500000000000000000, -1.299038105676658450, 17.69999999999999929 ) ) ;
#4409=ORIENTED_EDGE ( 'NONE', *, *, #4554, .F. ) ;
#4454=ORIENTED_EDGE ( 'NONE', *, *, #4301, .T. ) ;
#4458=DIRECTION ( 'NONE',  ( 0.000000000000000000, 0.000000000000000000, 1.000000000000000000 ) ) ;
#4465=EDGE_CURVE ( 'NONE', #4120, #4100, #3677, .T. ) ;
#4496=VERTEX_POINT ( 'NONE', #4407 ) ;
#4502=EDGE_CURVE ( 'NONE', #27, #2849, #2234, .T. ) ;
#4504=PRESENTATION_STYLE_ASSIGNMENT (( #1320 ) ) ;
#4512=CARTESIAN_POINT ( 'NONE',  ( 0.7500000000000000000, 0.000000000000000000, 17.69999999999999929 ) ) ;
#4554=EDGE_CURVE ( 'NONE', #788, #1550, #482, .T. ) ;
#4555=AXIS2_PLACEMENT_3D ( 'NONE', #3644, #435, #1886 ) ;
#4567=FACE_OUTER_BOUND ( 'NONE', #1820, .T. ) ;
#4574=CARTESIAN_POINT ( 'NONE',  ( 1.500000000000000222, 0.000000000000000000, 18.19999999999999929 ) ) ;
#4591=DIRECTION ( 'NONE',  ( 1.000000000000000000, 0.000000000000000000, 0.000000000000000000 ) ) ;
#4595=VERTEX_POINT ( 'NONE', #4180 ) ;
#4598=SURFACE_STYLE_FILL_AREA ( #2683 ) ;
#4603=DIRECTION ( 'NONE',  ( 1.000000000000000000, 0.000000000000000000, 0.000000000000000000 ) ) ;
#4608=DIRECTION ( 'NONE',  ( 0.000000000000000000, 0.000000000000000000, 1.000000000000000000 ) ) ;
#4616=DIRECTION ( 'NONE',  ( 1.000000000000000000, 0.000000000000000000, 0.000000000000000000 ) ) ;
#4622=EDGE_CURVE ( 'NONE', #1560, #2878, #1665, .T. ) ;
#4626=PRODUCT_DEFINITION_CONTEXT ( 'detailed design', #2515, 'design' ) ;
#4627=DIRECTION ( 'NONE',  ( 0.000000000000000000, 0.000000000000000000, 1.000000000000000000 ) ) ;
#4630=VECTOR ( 'NONE', #2459, 1000.000000000000000 ) ;
#4632=EDGE_LOOP ( 'NONE', ( #720, #449, #1071, #78 ) ) ;
#4675=EDGE_LOOP ( 'NONE', ( #1590, #2603, #3091, #1822 ) ) ;
#4677=DIRECTION ( 'NONE',  ( 0.000000000000000000, 0.000000000000000000, 1.000000000000000000 ) ) ;
#4682=AXIS2_PLACEMENT_3D ( 'NONE', #512, #3412, #3481 ) ;
#4688=PRODUCT_CONTEXT ( 'NONE', #2446, 'mechanical' ) ;
#4730=COLOUR_RGB('Sky Blue',0.24,0.69,0.87);
#4731=FILL_AREA_STYLE_COLOUR('',#4730);
#4732=FILL_AREA_STYLE('',(#4731));
#4733=SURFACE_STYLE_FILL_AREA(#4732);
#4734=SURFACE_SIDE_STYLE('',(#4733));
#4735=SURFACE_STYLE_USAGE(.BOTH.,#4734);
#4736=PRESENTATION_STYLE_ASSIGNMENT((#4735));
ENDSEC;
END-ISO-10303-21;
